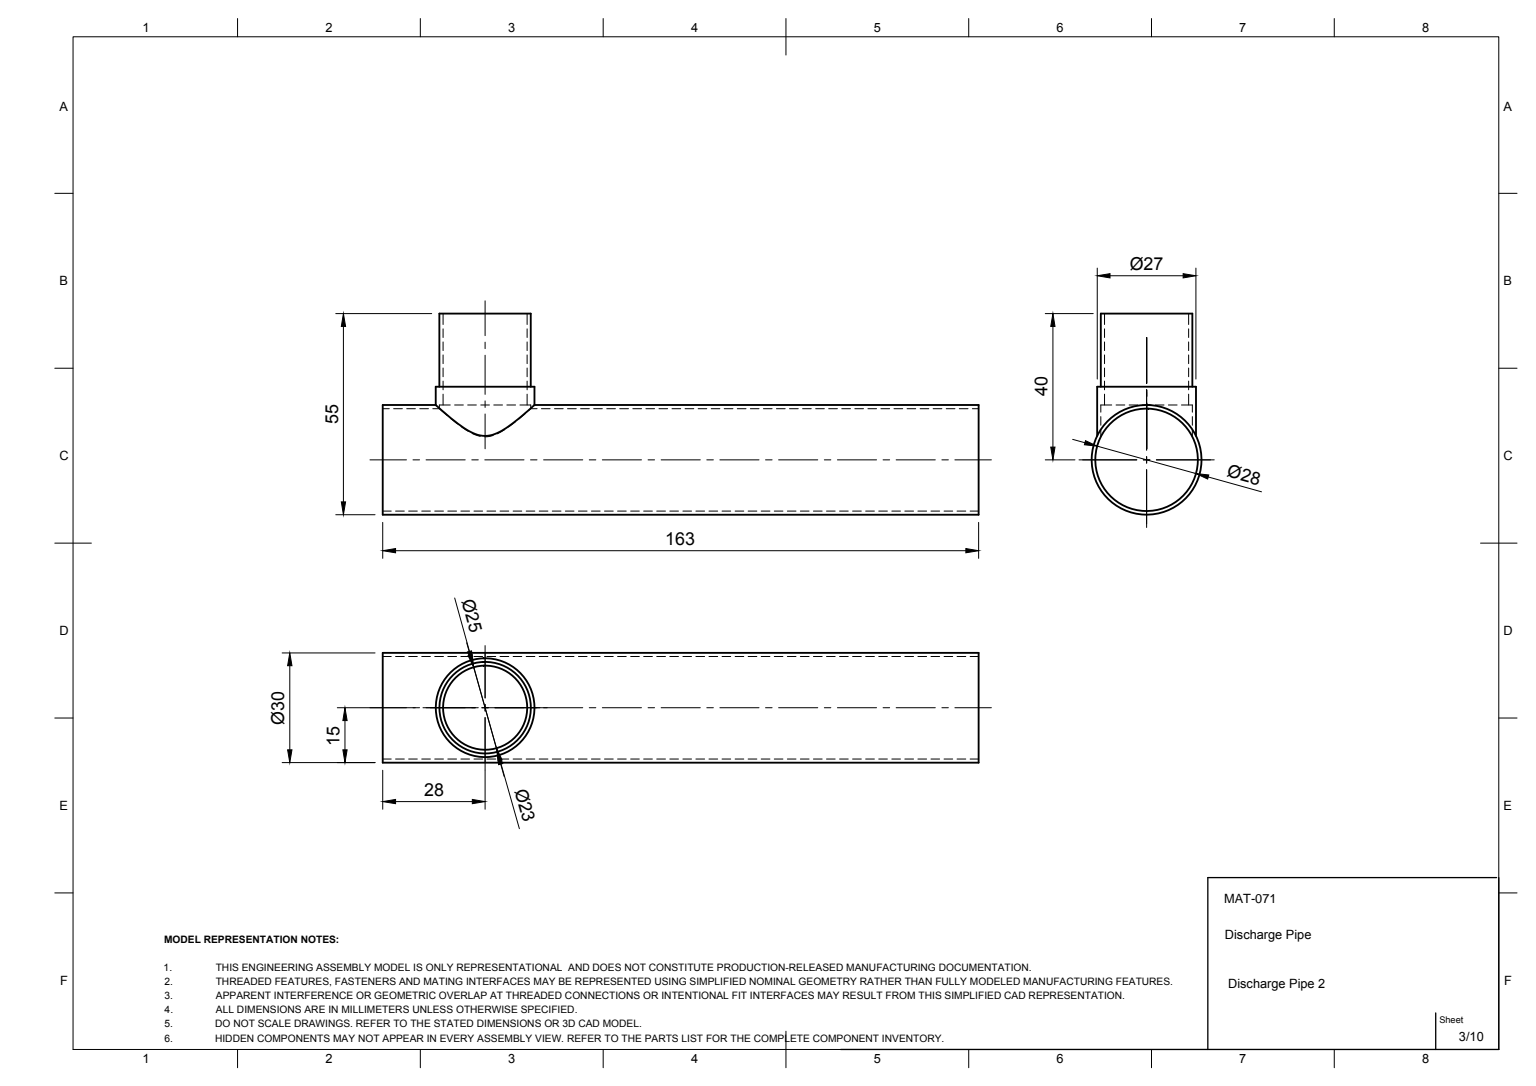
ISO-10303-21;
HEADER;
/* Generated by software containing ST-Developer
 * from STEP Tools, Inc. (www.steptools.com) 
 */

FILE_DESCRIPTION(
/* description */ (''),
/* implementation_level */ '2;1');

FILE_NAME(
/* name */ 'Discharge Pipe.step',
/* time_stamp */ '2026-10-24T12:24:47-07:00',
/* author */ (''),
/* organization */ (''),
/* preprocessor_version */ 'ST-DEVELOPER v20.2',
/* originating_system */ 'Autodesk Translation Framework v15.15.0.0',
/* authorisation */ '');

FILE_SCHEMA (('AUTOMOTIVE_DESIGN { 1 0 10303 214 3 1 1 }'));
ENDSEC;

DATA;
#10=MECHANICAL_DESIGN_GEOMETRIC_PRESENTATION_REPRESENTATION('',(#59),#13594);
#47=SHAPE_REPRESENTATION_RELATIONSHIP('SRR','None',#13627,#53);
#53=ADVANCED_BREP_SHAPE_REPRESENTATION('',(#65),#13590);
#59=STYLED_ITEM('',(#13667),#65);
#65=MANIFOLD_SOLID_BREP('Discharge Pipe 2',#2966);
#90=PLANE('',#3185);
#91=PLANE('',#3188);
#92=PLANE('',#3195);
#93=PLANE('',#3199);
#94=PLANE('',#3203);
#118=FACE_BOUND('',#508,.T.);
#119=FACE_BOUND('',#510,.T.);
#120=FACE_BOUND('',#512,.T.);
#121=FACE_BOUND('',#514,.T.);
#122=FACE_BOUND('',#517,.T.);
#123=FACE_BOUND('',#520,.T.);
#124=FACE_BOUND('',#523,.T.);
#139=B_SPLINE_CURVE_WITH_KNOTS('',3,(#11078,#11079,#11080,#11081,#11082,
#11083,#11084,#11085,#11086,#11087,#11088,#11089,#11090,#11091,#11092,#11093,
#11094,#11095,#11096,#11097,#11098,#11099,#11100,#11101,#11102,#11103,#11104,
#11105,#11106,#11107),.UNSPECIFIED.,.F.,.F.,(4,2,2,2,2,2,2,2,2,2,2,2,2,
2,4),(-4.18591455437331,-3.91515878973024,-3.64440302508717,-3.3736472604441,
-3.10289149580103,-2.59792438649385,-2.34544083184025,-2.09295727718666,
-1.84047372253307,-1.58799016787947,-1.08302305857229,-0.812267293929217,
-0.541511529286145,-0.270755764643072,0.),.UNSPECIFIED.);
#140=B_SPLINE_CURVE_WITH_KNOTS('',3,(#11108,#11109,#11110,#11111,#11112,
#11113,#11114,#11115,#11116,#11117,#11118,#11119,#11120,#11121,#11122,#11123,
#11124,#11125,#11126,#11127,#11128,#11129,#11130,#11131,#11132,#11133,#11134,
#11135,#11136,#11137),.UNSPECIFIED.,.F.,.F.,(4,2,2,2,2,2,2,2,2,2,2,2,2,
2,4),(0.,0.270755764643072,0.541511529286144,0.812267293929215,1.08302305857229,
1.58799016787947,1.84047372253307,2.09295727718666,2.34544083184025,2.59792438649385,
3.10289149580103,3.3736472604441,3.64440302508717,3.91515878973024,4.18591455437331),
 .UNSPECIFIED.);
#141=B_SPLINE_CURVE_WITH_KNOTS('',3,(#11155,#11156,#11157,#11158,#11159,
#11160,#11161,#11162,#11163,#11164,#11165,#11166,#11167,#11168,#11169,#11170,
#11171,#11172,#11173,#11174,#11175,#11176,#11177,#11178,#11179,#11180,#11181,
#11182,#11183,#11184),.UNSPECIFIED.,.F.,.F.,(4,2,2,2,2,2,2,2,2,2,2,2,2,
2,4),(4.53865697324691,4.83291964941679,5.12718232558667,5.42144500175655,
5.71570767792644,6.2618465688984,6.53491601438438,6.80798545987036,7.08105490535634,
7.35412435084232,7.90026324181428,8.19452591798416,8.48878859415405,8.78305127032393,
9.07731394649381),.UNSPECIFIED.);
#142=B_SPLINE_CURVE_WITH_KNOTS('',3,(#11185,#11186,#11187,#11188,#11189,
#11190,#11191,#11192,#11193,#11194,#11195,#11196,#11197,#11198,#11199,#11200,
#11201,#11202,#11203,#11204,#11205,#11206,#11207,#11208,#11209,#11210,#11211,
#11212,#11213,#11214),.UNSPECIFIED.,.F.,.F.,(4,2,2,2,2,2,2,2,2,2,2,2,2,
2,4),(9.07731394649381,9.3715766226637,9.66583929883358,9.96010197500346,
10.2543646511733,10.8005035421453,11.0735729876313,11.3466424331173,11.6197118786033,
11.8927813240892,12.4389202150612,12.7331828912311,13.027445567401,13.3217082435708,
13.6159709197407),.UNSPECIFIED.);
#166=CIRCLE('',#3184,12.5);
#167=CIRCLE('',#3186,15.);
#168=CIRCLE('',#3187,14.);
#169=CIRCLE('',#3189,15.);
#170=CIRCLE('',#3190,14.);
#171=CIRCLE('',#3194,13.5);
#172=CIRCLE('',#3196,12.5);
#173=CIRCLE('',#3198,12.5);
#174=CIRCLE('',#3200,11.5);
#175=CIRCLE('',#3202,11.5);
#330=FACE_OUTER_BOUND('',#506,.T.);
#331=FACE_OUTER_BOUND('',#507,.T.);
#332=FACE_OUTER_BOUND('',#509,.T.);
#333=FACE_OUTER_BOUND('',#511,.T.);
#334=FACE_OUTER_BOUND('',#513,.T.);
#335=FACE_OUTER_BOUND('',#515,.T.);
#336=FACE_OUTER_BOUND('',#516,.T.);
#337=FACE_OUTER_BOUND('',#518,.T.);
#338=FACE_OUTER_BOUND('',#519,.T.);
#339=FACE_OUTER_BOUND('',#521,.T.);
#340=FACE_OUTER_BOUND('',#522,.T.);
#506=EDGE_LOOP('',(#2487,#2488,#2489,#2490,#2491));
#507=EDGE_LOOP('',(#2492));
#508=EDGE_LOOP('',(#2493));
#509=EDGE_LOOP('',(#2494));
#510=EDGE_LOOP('',(#2495));
#511=EDGE_LOOP('',(#2496,#2497,#2498,#2499));
#512=EDGE_LOOP('',(#2500,#2501));
#513=EDGE_LOOP('',(#2502,#2503,#2504,#2505));
#514=EDGE_LOOP('',(#2506,#2507));
#515=EDGE_LOOP('',(#2508,#2509,#2510,#2511,#2512));
#516=EDGE_LOOP('',(#2513));
#517=EDGE_LOOP('',(#2514));
#518=EDGE_LOOP('',(#2515,#2516,#2517,#2518));
#519=EDGE_LOOP('',(#2519));
#520=EDGE_LOOP('',(#2520));
#521=EDGE_LOOP('',(#2521,#2522,#2523,#2524));
#522=EDGE_LOOP('',(#2525));
#523=EDGE_LOOP('',(#2526));
#897=LINE('',#11139,#1048);
#898=LINE('',#11152,#1049);
#899=LINE('',#11216,#1050);
#900=LINE('',#11220,#1051);
#901=LINE('',#11227,#1052);
#902=LINE('',#11233,#1053);
#1048=VECTOR('',#3687,12.5);
#1049=VECTOR('',#3704,15.);
#1050=VECTOR('',#3707,14.);
#1051=VECTOR('',#3712,13.5);
#1052=VECTOR('',#3721,12.5);
#1053=VECTOR('',#3728,11.5);
#1309=VERTEX_POINT('',#11076);
#1310=VERTEX_POINT('',#11077);
#1311=VERTEX_POINT('',#11138);
#1312=VERTEX_POINT('',#11142);
#1313=VERTEX_POINT('',#11144);
#1314=VERTEX_POINT('',#11147);
#1315=VERTEX_POINT('',#11149);
#1316=VERTEX_POINT('',#11153);
#1317=VERTEX_POINT('',#11154);
#1318=VERTEX_POINT('',#11218);
#1319=VERTEX_POINT('',#11222);
#1320=VERTEX_POINT('',#11225);
#1321=VERTEX_POINT('',#11229);
#1322=VERTEX_POINT('',#11232);
#1712=EDGE_CURVE('',#1309,#1310,#139,.T.);
#1713=EDGE_CURVE('',#1310,#1309,#140,.T.);
#1714=EDGE_CURVE('',#1310,#1311,#897,.T.);
#1715=EDGE_CURVE('',#1311,#1311,#166,.F.);
#1716=EDGE_CURVE('',#1312,#1312,#167,.T.);
#1717=EDGE_CURVE('',#1313,#1313,#168,.T.);
#1718=EDGE_CURVE('',#1314,#1314,#169,.T.);
#1719=EDGE_CURVE('',#1315,#1315,#170,.T.);
#1720=EDGE_CURVE('',#1314,#1312,#898,.T.);
#1721=EDGE_CURVE('',#1316,#1317,#141,.T.);
#1722=EDGE_CURVE('',#1317,#1316,#142,.T.);
#1723=EDGE_CURVE('',#1313,#1315,#899,.T.);
#1724=EDGE_CURVE('',#1318,#1318,#171,.T.);
#1725=EDGE_CURVE('',#1318,#1317,#900,.T.);
#1726=EDGE_CURVE('',#1319,#1319,#172,.T.);
#1727=EDGE_CURVE('',#1320,#1320,#173,.T.);
#1728=EDGE_CURVE('',#1320,#1319,#901,.T.);
#1729=EDGE_CURVE('',#1321,#1321,#174,.T.);
#1730=EDGE_CURVE('',#1321,#1322,#902,.T.);
#1731=EDGE_CURVE('',#1322,#1322,#175,.T.);
#2487=ORIENTED_EDGE('',*,*,#1712,.F.);
#2488=ORIENTED_EDGE('',*,*,#1713,.F.);
#2489=ORIENTED_EDGE('',*,*,#1714,.T.);
#2490=ORIENTED_EDGE('',*,*,#1715,.F.);
#2491=ORIENTED_EDGE('',*,*,#1714,.F.);
#2492=ORIENTED_EDGE('',*,*,#1716,.F.);
#2493=ORIENTED_EDGE('',*,*,#1717,.T.);
#2494=ORIENTED_EDGE('',*,*,#1718,.T.);
#2495=ORIENTED_EDGE('',*,*,#1719,.F.);
#2496=ORIENTED_EDGE('',*,*,#1718,.F.);
#2497=ORIENTED_EDGE('',*,*,#1720,.T.);
#2498=ORIENTED_EDGE('',*,*,#1716,.T.);
#2499=ORIENTED_EDGE('',*,*,#1720,.F.);
#2500=ORIENTED_EDGE('',*,*,#1721,.F.);
#2501=ORIENTED_EDGE('',*,*,#1722,.F.);
#2502=ORIENTED_EDGE('',*,*,#1717,.F.);
#2503=ORIENTED_EDGE('',*,*,#1723,.T.);
#2504=ORIENTED_EDGE('',*,*,#1719,.T.);
#2505=ORIENTED_EDGE('',*,*,#1723,.F.);
#2506=ORIENTED_EDGE('',*,*,#1712,.T.);
#2507=ORIENTED_EDGE('',*,*,#1713,.T.);
#2508=ORIENTED_EDGE('',*,*,#1724,.F.);
#2509=ORIENTED_EDGE('',*,*,#1725,.T.);
#2510=ORIENTED_EDGE('',*,*,#1722,.T.);
#2511=ORIENTED_EDGE('',*,*,#1721,.T.);
#2512=ORIENTED_EDGE('',*,*,#1725,.F.);
#2513=ORIENTED_EDGE('',*,*,#1724,.T.);
#2514=ORIENTED_EDGE('',*,*,#1726,.F.);
#2515=ORIENTED_EDGE('',*,*,#1727,.F.);
#2516=ORIENTED_EDGE('',*,*,#1728,.T.);
#2517=ORIENTED_EDGE('',*,*,#1726,.T.);
#2518=ORIENTED_EDGE('',*,*,#1728,.F.);
#2519=ORIENTED_EDGE('',*,*,#1715,.T.);
#2520=ORIENTED_EDGE('',*,*,#1729,.T.);
#2521=ORIENTED_EDGE('',*,*,#1729,.F.);
#2522=ORIENTED_EDGE('',*,*,#1730,.T.);
#2523=ORIENTED_EDGE('',*,*,#1731,.T.);
#2524=ORIENTED_EDGE('',*,*,#1730,.F.);
#2525=ORIENTED_EDGE('',*,*,#1727,.T.);
#2526=ORIENTED_EDGE('',*,*,#1731,.F.);
#2776=CYLINDRICAL_SURFACE('',#3183,12.5);
#2777=CYLINDRICAL_SURFACE('',#3191,15.);
#2778=CYLINDRICAL_SURFACE('',#3192,14.);
#2779=CYLINDRICAL_SURFACE('',#3193,13.5);
#2780=CYLINDRICAL_SURFACE('',#3197,12.5);
#2781=CYLINDRICAL_SURFACE('',#3201,11.5);
#2917=ADVANCED_FACE('',(#330),#2776,.F.);
#2918=ADVANCED_FACE('',(#331,#118),#90,.F.);
#2919=ADVANCED_FACE('',(#332,#119),#91,.T.);
#2920=ADVANCED_FACE('',(#333,#120),#2777,.T.);
#2921=ADVANCED_FACE('',(#334,#121),#2778,.F.);
#2922=ADVANCED_FACE('',(#335),#2779,.T.);
#2923=ADVANCED_FACE('',(#336,#122),#92,.T.);
#2924=ADVANCED_FACE('',(#337),#2780,.T.);
#2925=ADVANCED_FACE('',(#338,#123),#93,.F.);
#2926=ADVANCED_FACE('',(#339),#2781,.F.);
#2927=ADVANCED_FACE('',(#340,#124),#94,.T.);
#2966=CLOSED_SHELL('',(#2917,#2918,#2919,#2920,#2921,#2922,#2923,#2924,
#2925,#2926,#2927));
#3182=AXIS2_PLACEMENT_3D('',#11074,#3683,#3684);
#3183=AXIS2_PLACEMENT_3D('',#11075,#3685,#3686);
#3184=AXIS2_PLACEMENT_3D('',#11140,#3688,#3689);
#3185=AXIS2_PLACEMENT_3D('',#11141,#3690,#3691);
#3186=AXIS2_PLACEMENT_3D('',#11143,#3692,#3693);
#3187=AXIS2_PLACEMENT_3D('',#11145,#3694,#3695);
#3188=AXIS2_PLACEMENT_3D('',#11146,#3696,#3697);
#3189=AXIS2_PLACEMENT_3D('',#11148,#3698,#3699);
#3190=AXIS2_PLACEMENT_3D('',#11150,#3700,#3701);
#3191=AXIS2_PLACEMENT_3D('',#11151,#3702,#3703);
#3192=AXIS2_PLACEMENT_3D('',#11215,#3705,#3706);
#3193=AXIS2_PLACEMENT_3D('',#11217,#3708,#3709);
#3194=AXIS2_PLACEMENT_3D('',#11219,#3710,#3711);
#3195=AXIS2_PLACEMENT_3D('',#11221,#3713,#3714);
#3196=AXIS2_PLACEMENT_3D('',#11223,#3715,#3716);
#3197=AXIS2_PLACEMENT_3D('',#11224,#3717,#3718);
#3198=AXIS2_PLACEMENT_3D('',#11226,#3719,#3720);
#3199=AXIS2_PLACEMENT_3D('',#11228,#3722,#3723);
#3200=AXIS2_PLACEMENT_3D('',#11230,#3724,#3725);
#3201=AXIS2_PLACEMENT_3D('',#11231,#3726,#3727);
#3202=AXIS2_PLACEMENT_3D('',#11234,#3729,#3730);
#3203=AXIS2_PLACEMENT_3D('',#11235,#3731,#3732);
#3683=DIRECTION('axis',(0.,0.,1.));
#3684=DIRECTION('refdir',(1.,0.,0.));
#3685=DIRECTION('center_axis',(1.73472347597681E-16,1.,0.));
#3686=DIRECTION('ref_axis',(-1.,1.73472347597681E-16,0.));
#3687=DIRECTION('',(1.73472347597681E-16,1.,0.));
#3688=DIRECTION('center_axis',(1.73472347597681E-16,1.,0.));
#3689=DIRECTION('ref_axis',(-1.,1.73472347597681E-16,0.));
#3690=DIRECTION('center_axis',(0.,0.,-1.));
#3691=DIRECTION('ref_axis',(-1.,0.,0.));
#3692=DIRECTION('center_axis',(0.,0.,-1.));
#3693=DIRECTION('ref_axis',(-1.,0.,0.));
#3694=DIRECTION('center_axis',(0.,0.,-1.));
#3695=DIRECTION('ref_axis',(-1.,0.,0.));
#3696=DIRECTION('center_axis',(0.,0.,-1.));
#3697=DIRECTION('ref_axis',(-1.,0.,0.));
#3698=DIRECTION('center_axis',(0.,0.,-1.));
#3699=DIRECTION('ref_axis',(-1.,0.,0.));
#3700=DIRECTION('center_axis',(0.,0.,-1.));
#3701=DIRECTION('ref_axis',(-1.,0.,0.));
#3702=DIRECTION('center_axis',(0.,0.,-1.));
#3703=DIRECTION('ref_axis',(-1.,0.,0.));
#3704=DIRECTION('',(0.,0.,1.));
#3705=DIRECTION('center_axis',(0.,0.,-1.));
#3706=DIRECTION('ref_axis',(-1.,0.,0.));
#3707=DIRECTION('',(0.,0.,-1.));
#3708=DIRECTION('center_axis',(1.73472347597681E-16,1.,0.));
#3709=DIRECTION('ref_axis',(-1.,1.73472347597681E-16,0.));
#3710=DIRECTION('center_axis',(1.73472347597681E-16,1.,0.));
#3711=DIRECTION('ref_axis',(-1.,1.73472347597681E-16,0.));
#3712=DIRECTION('',(-1.73472347597681E-16,-1.,0.));
#3713=DIRECTION('center_axis',(1.73472347597681E-16,1.,0.));
#3714=DIRECTION('ref_axis',(0.,0.,1.));
#3715=DIRECTION('center_axis',(1.73472347597681E-16,1.,0.));
#3716=DIRECTION('ref_axis',(1.,-1.73472347597681E-16,0.));
#3717=DIRECTION('center_axis',(1.73472347597681E-16,1.,0.));
#3718=DIRECTION('ref_axis',(-1.,1.73472347597681E-16,0.));
#3719=DIRECTION('center_axis',(1.73472347597681E-16,1.,0.));
#3720=DIRECTION('ref_axis',(-1.,1.73472347597681E-16,0.));
#3721=DIRECTION('',(-1.73472347597681E-16,-1.,0.));
#3722=DIRECTION('center_axis',(1.73472347597681E-16,1.,0.));
#3723=DIRECTION('ref_axis',(0.,0.,1.));
#3724=DIRECTION('center_axis',(1.73472347597681E-16,1.,0.));
#3725=DIRECTION('ref_axis',(1.,-1.73472347597681E-16,0.));
#3726=DIRECTION('center_axis',(1.73472347597681E-16,1.,0.));
#3727=DIRECTION('ref_axis',(-1.,1.73472347597681E-16,0.));
#3728=DIRECTION('',(1.73472347597681E-16,1.,0.));
#3729=DIRECTION('center_axis',(1.73472347597681E-16,1.,0.));
#3730=DIRECTION('ref_axis',(1.,-1.73472347597681E-16,0.));
#3731=DIRECTION('center_axis',(1.73472347597681E-16,1.,0.));
#3732=DIRECTION('ref_axis',(0.,0.,1.));
#11074=CARTESIAN_POINT('',(0.,0.,0.));
#11075=CARTESIAN_POINT('Origin',(-6.07016839548973E-14,-537.001,260.5));
#11076=CARTESIAN_POINT('',(-12.5,6.3047601064593,260.5));
#11077=CARTESIAN_POINT('',(12.5,6.30476010645914,260.5));
#11078=CARTESIAN_POINT('Ctrl Pts',(-12.5,6.30476010645931,260.5));
#11079=CARTESIAN_POINT('Ctrl Pts',(-12.5,6.30476010645931,261.402519215477));
#11080=CARTESIAN_POINT('Ctrl Pts',(-12.4043127929448,6.50044843544715,262.252785687934));
#11081=CARTESIAN_POINT('Ctrl Pts',(-12.0635561086719,7.11290498732527,263.87784696441));
#11082=CARTESIAN_POINT('Ctrl Pts',(-11.8174017497439,7.5270600588976,264.653397811714));
#11083=CARTESIAN_POINT('Ctrl Pts',(-11.1849437511818,8.43828057198777,266.139053437606));
#11084=CARTESIAN_POINT('Ctrl Pts',(-10.798286104564,8.93532092407379,266.84711374057));
#11085=CARTESIAN_POINT('Ctrl Pts',(-9.90196102753225,9.91938057635149,268.170723777041));
#11086=CARTESIAN_POINT('Ctrl Pts',(-9.39191602949771,10.4067552745245,268.785753500166));
#11087=CARTESIAN_POINT('Ctrl Pts',(-7.80732266462415,11.6967917658663,270.370346865039));
#11088=CARTESIAN_POINT('Ctrl Pts',(-6.47055303401493,12.5222310217994,271.323893855586));
#11089=CARTESIAN_POINT('Ctrl Pts',(-4.17535648184543,13.3878671232299,272.311438876291));
#11090=CARTESIAN_POINT('Ctrl Pts',(-3.36242380893801,13.6166122026276,272.569314105635));
#11091=CARTESIAN_POINT('Ctrl Pts',(-1.69558088010183,13.9227521430804,272.913671589856));
#11092=CARTESIAN_POINT('Ctrl Pts',(-0.841611848845278,14.,273.));
#11093=CARTESIAN_POINT('Ctrl Pts',(0.841611848845341,14.,273.));
#11094=CARTESIAN_POINT('Ctrl Pts',(1.69558088010189,13.9227521430804,272.913671589856));
#11095=CARTESIAN_POINT('Ctrl Pts',(3.36242380893806,13.6166122026275,272.569314105635));
#11096=CARTESIAN_POINT('Ctrl Pts',(4.17535648184549,13.3878671232299,272.311438876291));
#11097=CARTESIAN_POINT('Ctrl Pts',(6.47055303401499,12.5222310217993,271.323893855586));
#11098=CARTESIAN_POINT('Ctrl Pts',(7.80732266462421,11.6967917658663,270.370346865039));
#11099=CARTESIAN_POINT('Ctrl Pts',(9.39191602949777,10.4067552745245,268.785753500166));
#11100=CARTESIAN_POINT('Ctrl Pts',(9.9019610275323,9.91938057635144,268.170723777041));
#11101=CARTESIAN_POINT('Ctrl Pts',(10.7982861045641,8.93532092407374,266.84711374057));
#11102=CARTESIAN_POINT('Ctrl Pts',(11.1849437511818,8.4382805719877,266.139053437606));
#11103=CARTESIAN_POINT('Ctrl Pts',(11.817401749744,7.5270600588975,264.653397811714));
#11104=CARTESIAN_POINT('Ctrl Pts',(12.063556108672,7.11290498732516,263.87784696441));
#11105=CARTESIAN_POINT('Ctrl Pts',(12.4043127929449,6.50044843544704,262.252785687934));
#11106=CARTESIAN_POINT('Ctrl Pts',(12.5,6.30476010645918,261.402519215477));
#11107=CARTESIAN_POINT('Ctrl Pts',(12.5,6.30476010645918,260.5));
#11108=CARTESIAN_POINT('Ctrl Pts',(12.5,6.30476010645918,260.5));
#11109=CARTESIAN_POINT('Ctrl Pts',(12.5,6.30476010645918,259.597480784523));
#11110=CARTESIAN_POINT('Ctrl Pts',(12.4043127929449,6.50044843544704,258.747214312066));
#11111=CARTESIAN_POINT('Ctrl Pts',(12.063556108672,7.11290498732516,257.12215303559));
#11112=CARTESIAN_POINT('Ctrl Pts',(11.817401749744,7.5270600588975,256.346602188286));
#11113=CARTESIAN_POINT('Ctrl Pts',(11.1849437511818,8.4382805719877,254.860946562394));
#11114=CARTESIAN_POINT('Ctrl Pts',(10.7982861045641,8.93532092407371,254.15288625943));
#11115=CARTESIAN_POINT('Ctrl Pts',(9.90196102753233,9.91938057635141,252.829276222959));
#11116=CARTESIAN_POINT('Ctrl Pts',(9.39191602949779,10.4067552745245,252.214246499834));
#11117=CARTESIAN_POINT('Ctrl Pts',(7.80732266462423,11.6967917658663,250.629653134961));
#11118=CARTESIAN_POINT('Ctrl Pts',(6.47055303401501,12.5222310217993,249.676106144414));
#11119=CARTESIAN_POINT('Ctrl Pts',(4.17535648184551,13.3878671232299,248.688561123709));
#11120=CARTESIAN_POINT('Ctrl Pts',(3.36242380893808,13.6166122026275,248.430685894365));
#11121=CARTESIAN_POINT('Ctrl Pts',(1.6955808801019,13.9227521430804,248.086328410144));
#11122=CARTESIAN_POINT('Ctrl Pts',(0.841611848845347,14.,248.));
#11123=CARTESIAN_POINT('Ctrl Pts',(-0.841611848845273,14.,248.));
#11124=CARTESIAN_POINT('Ctrl Pts',(-1.69558088010183,13.9227521430804,248.086328410144));
#11125=CARTESIAN_POINT('Ctrl Pts',(-3.362423808938,13.6166122026276,248.430685894365));
#11126=CARTESIAN_POINT('Ctrl Pts',(-4.17535648184543,13.3878671232299,248.688561123709));
#11127=CARTESIAN_POINT('Ctrl Pts',(-6.47055303401493,12.5222310217994,249.676106144414));
#11128=CARTESIAN_POINT('Ctrl Pts',(-7.80732266462415,11.6967917658663,250.629653134961));
#11129=CARTESIAN_POINT('Ctrl Pts',(-9.39191602949771,10.4067552745245,252.214246499834));
#11130=CARTESIAN_POINT('Ctrl Pts',(-9.90196102753228,9.91938057635146,252.829276222959));
#11131=CARTESIAN_POINT('Ctrl Pts',(-10.7982861045641,8.93532092407377,254.15288625943));
#11132=CARTESIAN_POINT('Ctrl Pts',(-11.1849437511818,8.43828057198777,254.860946562394));
#11133=CARTESIAN_POINT('Ctrl Pts',(-11.8174017497439,7.5270600588976,256.346602188286));
#11134=CARTESIAN_POINT('Ctrl Pts',(-12.0635561086719,7.11290498732527,257.122153035591));
#11135=CARTESIAN_POINT('Ctrl Pts',(-12.4043127929448,6.50044843544715,258.747214312066));
#11136=CARTESIAN_POINT('Ctrl Pts',(-12.5,6.30476010645931,259.597480784523));
#11137=CARTESIAN_POINT('Ctrl Pts',(-12.5,6.30476010645931,260.5));
#11138=CARTESIAN_POINT('',(12.5,15.,260.5));
#11139=CARTESIAN_POINT('',(12.4999999999999,-537.001,260.5));
#11140=CARTESIAN_POINT('Origin',(3.50552253913701E-14,15.,260.5));
#11141=CARTESIAN_POINT('Origin',(0.,0.,288.5));
#11142=CARTESIAN_POINT('',(15.,-1.83697019872103E-15,288.5));
#11143=CARTESIAN_POINT('Origin',(0.,0.,288.5));
#11144=CARTESIAN_POINT('',(14.,-1.71450551880629E-15,288.5));
#11145=CARTESIAN_POINT('Origin',(0.,0.,288.5));
#11146=CARTESIAN_POINT('Origin',(0.,0.,125.5));
#11147=CARTESIAN_POINT('',(15.,-1.83697019872103E-15,125.5));
#11148=CARTESIAN_POINT('Origin',(0.,0.,125.5));
#11149=CARTESIAN_POINT('',(14.,-1.71450551880629E-15,125.5));
#11150=CARTESIAN_POINT('Origin',(0.,0.,125.5));
#11151=CARTESIAN_POINT('Origin',(0.,0.,288.5));
#11152=CARTESIAN_POINT('',(15.,-1.83697019872103E-15,288.5));
#11153=CARTESIAN_POINT('',(-13.5,6.53834841531107,260.5));
#11154=CARTESIAN_POINT('',(13.5,6.53834841531101,260.5));
#11155=CARTESIAN_POINT('Ctrl Pts',(-13.5,6.53834841531108,260.5));
#11156=CARTESIAN_POINT('Ctrl Pts',(-13.5,6.53834841531108,261.480875587233));
#11157=CARTESIAN_POINT('Ctrl Pts',(-13.3958232026777,6.76037527468857,262.398034825266));
#11158=CARTESIAN_POINT('Ctrl Pts',(-13.0281423324427,7.44434384956079,264.149401104853));
#11159=CARTESIAN_POINT('Ctrl Pts',(-12.7631917195318,7.9038410644566,264.984257909941));
#11160=CARTESIAN_POINT('Ctrl Pts',(-12.0815890679171,8.91094016019654,266.586308189152));
#11161=CARTESIAN_POINT('Ctrl Pts',(-11.6646347002389,9.45851405605539,267.350709749346));
#11162=CARTESIAN_POINT('Ctrl Pts',(-10.6965567278803,10.5409138836385,268.78128013682));
#11163=CARTESIAN_POINT('Ctrl Pts',(-10.1450315382585,11.0761700594821,269.446851553778));
#11164=CARTESIAN_POINT('Ctrl Pts',(-8.43405624607796,12.487773690397,271.157826845959));
#11165=CARTESIAN_POINT('Ctrl Pts',(-6.99182923331508,13.388092684802,272.187651131601));
#11166=CARTESIAN_POINT('Ctrl Pts',(-4.51318011101059,14.332232492506,273.255015840138));
#11167=CARTESIAN_POINT('Ctrl Pts',(-3.63493173087046,14.5817163893703,273.533927767516));
#11168=CARTESIAN_POINT('Ctrl Pts',(-1.83348931439436,14.9156796189506,273.906502850605));
#11169=CARTESIAN_POINT('Ctrl Pts',(-0.910231484953233,15.,274.));
#11170=CARTESIAN_POINT('Ctrl Pts',(0.910231484953305,15.,274.));
#11171=CARTESIAN_POINT('Ctrl Pts',(1.83348931439444,14.9156796189506,273.906502850605));
#11172=CARTESIAN_POINT('Ctrl Pts',(3.63493173087052,14.5817163893703,273.533927767516));
#11173=CARTESIAN_POINT('Ctrl Pts',(4.51318011101065,14.332232492506,273.255015840138));
#11174=CARTESIAN_POINT('Ctrl Pts',(6.99182923331514,13.3880926848019,272.187651131601));
#11175=CARTESIAN_POINT('Ctrl Pts',(8.43405624607803,12.4877736903969,271.157826845959));
#11176=CARTESIAN_POINT('Ctrl Pts',(10.1450315382585,11.0761700594821,269.446851553778));
#11177=CARTESIAN_POINT('Ctrl Pts',(10.6965567278803,10.5409138836385,268.78128013682));
#11178=CARTESIAN_POINT('Ctrl Pts',(11.664634700239,9.45851405605531,267.350709749346));
#11179=CARTESIAN_POINT('Ctrl Pts',(12.0815890679171,8.91094016019645,266.586308189152));
#11180=CARTESIAN_POINT('Ctrl Pts',(12.7631917195319,7.90384106445649,264.984257909941));
#11181=CARTESIAN_POINT('Ctrl Pts',(13.0281423324427,7.44434384956068,264.149401104853));
#11182=CARTESIAN_POINT('Ctrl Pts',(13.3958232026778,6.76037527468845,262.398034825266));
#11183=CARTESIAN_POINT('Ctrl Pts',(13.5,6.53834841531094,261.480875587233));
#11184=CARTESIAN_POINT('Ctrl Pts',(13.5,6.53834841531094,260.5));
#11185=CARTESIAN_POINT('Ctrl Pts',(13.5,6.53834841531094,260.5));
#11186=CARTESIAN_POINT('Ctrl Pts',(13.5,6.53834841531094,259.519124412767));
#11187=CARTESIAN_POINT('Ctrl Pts',(13.3958232026778,6.76037527468844,258.601965174734));
#11188=CARTESIAN_POINT('Ctrl Pts',(13.0281423324427,7.44434384956067,256.850598895147));
#11189=CARTESIAN_POINT('Ctrl Pts',(12.7631917195319,7.90384106445648,256.015742090059));
#11190=CARTESIAN_POINT('Ctrl Pts',(12.0815890679171,8.91094016019645,254.413691810848));
#11191=CARTESIAN_POINT('Ctrl Pts',(11.664634700239,9.4585140560553,253.649290250654));
#11192=CARTESIAN_POINT('Ctrl Pts',(10.6965567278803,10.5409138836385,252.21871986318));
#11193=CARTESIAN_POINT('Ctrl Pts',(10.1450315382585,11.0761700594821,251.553148446222));
#11194=CARTESIAN_POINT('Ctrl Pts',(8.43405624607803,12.4877736903969,249.842173154041));
#11195=CARTESIAN_POINT('Ctrl Pts',(6.99182923331515,13.3880926848019,248.812348868399));
#11196=CARTESIAN_POINT('Ctrl Pts',(4.51318011101067,14.332232492506,247.744984159862));
#11197=CARTESIAN_POINT('Ctrl Pts',(3.63493173087054,14.5817163893703,247.466072232484));
#11198=CARTESIAN_POINT('Ctrl Pts',(1.83348931439444,14.9156796189506,247.093497149395));
#11199=CARTESIAN_POINT('Ctrl Pts',(0.910231484953304,15.,247.));
#11200=CARTESIAN_POINT('Ctrl Pts',(-0.910231484953234,15.,247.));
#11201=CARTESIAN_POINT('Ctrl Pts',(-1.83348931439437,14.9156796189506,247.093497149395));
#11202=CARTESIAN_POINT('Ctrl Pts',(-3.63493173087047,14.5817163893703,247.466072232484));
#11203=CARTESIAN_POINT('Ctrl Pts',(-4.51318011101059,14.332232492506,247.744984159862));
#11204=CARTESIAN_POINT('Ctrl Pts',(-6.99182923331508,13.388092684802,248.812348868399));
#11205=CARTESIAN_POINT('Ctrl Pts',(-8.43405624607796,12.487773690397,249.842173154041));
#11206=CARTESIAN_POINT('Ctrl Pts',(-10.1450315382585,11.0761700594821,251.553148446222));
#11207=CARTESIAN_POINT('Ctrl Pts',(-10.6965567278803,10.5409138836385,252.21871986318));
#11208=CARTESIAN_POINT('Ctrl Pts',(-11.6646347002389,9.45851405605539,253.649290250654));
#11209=CARTESIAN_POINT('Ctrl Pts',(-12.0815890679171,8.91094016019654,254.413691810848));
#11210=CARTESIAN_POINT('Ctrl Pts',(-12.7631917195318,7.9038410644566,256.015742090059));
#11211=CARTESIAN_POINT('Ctrl Pts',(-13.0281423324427,7.44434384956078,256.850598895147));
#11212=CARTESIAN_POINT('Ctrl Pts',(-13.3958232026777,6.76037527468857,258.601965174734));
#11213=CARTESIAN_POINT('Ctrl Pts',(-13.5,6.53834841531108,259.519124412767));
#11214=CARTESIAN_POINT('Ctrl Pts',(-13.5,6.53834841531108,260.5));
#11215=CARTESIAN_POINT('Origin',(0.,0.,288.5));
#11216=CARTESIAN_POINT('',(14.,-1.71450551880629E-15,288.5));
#11217=CARTESIAN_POINT('Origin',(-6.07016839548973E-14,-537.001,260.5));
#11218=CARTESIAN_POINT('',(13.5,20.,260.5));
#11219=CARTESIAN_POINT('Origin',(3.59225871293585E-14,20.,260.5));
#11220=CARTESIAN_POINT('',(13.4999999999999,-537.001,260.5));
#11221=CARTESIAN_POINT('Origin',(3.59225871293585E-14,20.,260.5));
#11222=CARTESIAN_POINT('',(12.5,20.,260.5));
#11223=CARTESIAN_POINT('Origin',(3.59225871293585E-14,20.,260.5));
#11224=CARTESIAN_POINT('Origin',(3.50552253913701E-14,15.,260.5));
#11225=CARTESIAN_POINT('',(12.5,40.,260.5));
#11226=CARTESIAN_POINT('Origin',(3.93920340813121E-14,40.,260.5));
#11227=CARTESIAN_POINT('',(12.5,15.,260.5));
#11228=CARTESIAN_POINT('Origin',(3.50552253913701E-14,15.,260.5));
#11229=CARTESIAN_POINT('',(11.5,15.,260.5));
#11230=CARTESIAN_POINT('Origin',(3.50552253913701E-14,15.,260.5));
#11231=CARTESIAN_POINT('Origin',(3.50552253913701E-14,15.,260.5));
#11232=CARTESIAN_POINT('',(11.5,40.,260.5));
#11233=CARTESIAN_POINT('',(11.5,15.,260.5));
#11234=CARTESIAN_POINT('Origin',(3.93920340813121E-14,40.,260.5));
#11235=CARTESIAN_POINT('Origin',(3.93920340813121E-14,40.,260.5));
#13581=UNCERTAINTY_MEASURE_WITH_UNIT(LENGTH_MEASURE(0.01),#13595,
'DISTANCE_ACCURACY_VALUE',
'Maximum model space distance between geometric entities at asserted c
onnectivities');
#13585=UNCERTAINTY_MEASURE_WITH_UNIT(LENGTH_MEASURE(0.01),#13595,
'DISTANCE_ACCURACY_VALUE',
'Maximum model space distance between geometric entities at asserted c
onnectivities');
#13590=(
GEOMETRIC_REPRESENTATION_CONTEXT(3)
GLOBAL_UNCERTAINTY_ASSIGNED_CONTEXT((#13581))
GLOBAL_UNIT_ASSIGNED_CONTEXT((#13595,#13597,#13598))
REPRESENTATION_CONTEXT('','3D')
);
#13594=(
GEOMETRIC_REPRESENTATION_CONTEXT(3)
GLOBAL_UNCERTAINTY_ASSIGNED_CONTEXT((#13585))
GLOBAL_UNIT_ASSIGNED_CONTEXT((#13595,#13597,#13598))
REPRESENTATION_CONTEXT('','3D')
);
#13595=(
LENGTH_UNIT()
NAMED_UNIT(*)
SI_UNIT(.MILLI.,.METRE.)
);
#13597=(
NAMED_UNIT(*)
PLANE_ANGLE_UNIT()
SI_UNIT($,.RADIAN.)
);
#13598=(
NAMED_UNIT(*)
SI_UNIT($,.STERADIAN.)
SOLID_ANGLE_UNIT()
);
#13603=SHAPE_DEFINITION_REPRESENTATION(#13614,#13627);
#13614=PRODUCT_DEFINITION_SHAPE('',$,#13636);
#13627=SHAPE_REPRESENTATION('',(#3182),#13590);
#13631=PRODUCT_DEFINITION_CONTEXT('part definition',#13657,'design');
#13636=PRODUCT_DEFINITION('Discharge Pipe','Discharge Pipe',#13644,#13631);
#13644=PRODUCT_DEFINITION_FORMATION('',$,#13663);
#13657=APPLICATION_CONTEXT(
'Core Data for Automotive Mechanical Design Process');
#13658=PRODUCT_CONTEXT('part definition',#13657,'mechanical');
#13663=PRODUCT('Discharge Pipe','Discharge Pipe',$,(#13658));
#13667=PRESENTATION_STYLE_ASSIGNMENT((#13668));
#13668=SURFACE_STYLE_USAGE(.BOTH.,#13669);
#13669=SURFACE_SIDE_STYLE('',(#13670));
#13670=SURFACE_STYLE_FILL_AREA(#13671);
#13671=FILL_AREA_STYLE('Steel - Satin',(#13672));
#13672=FILL_AREA_STYLE_COLOUR('Steel - Satin',#13673);
#13673=COLOUR_RGB('Steel - Satin',0.627450980392157,0.627450980392157,0.627450980392157);
ENDSEC;
END-ISO-10303-21;
